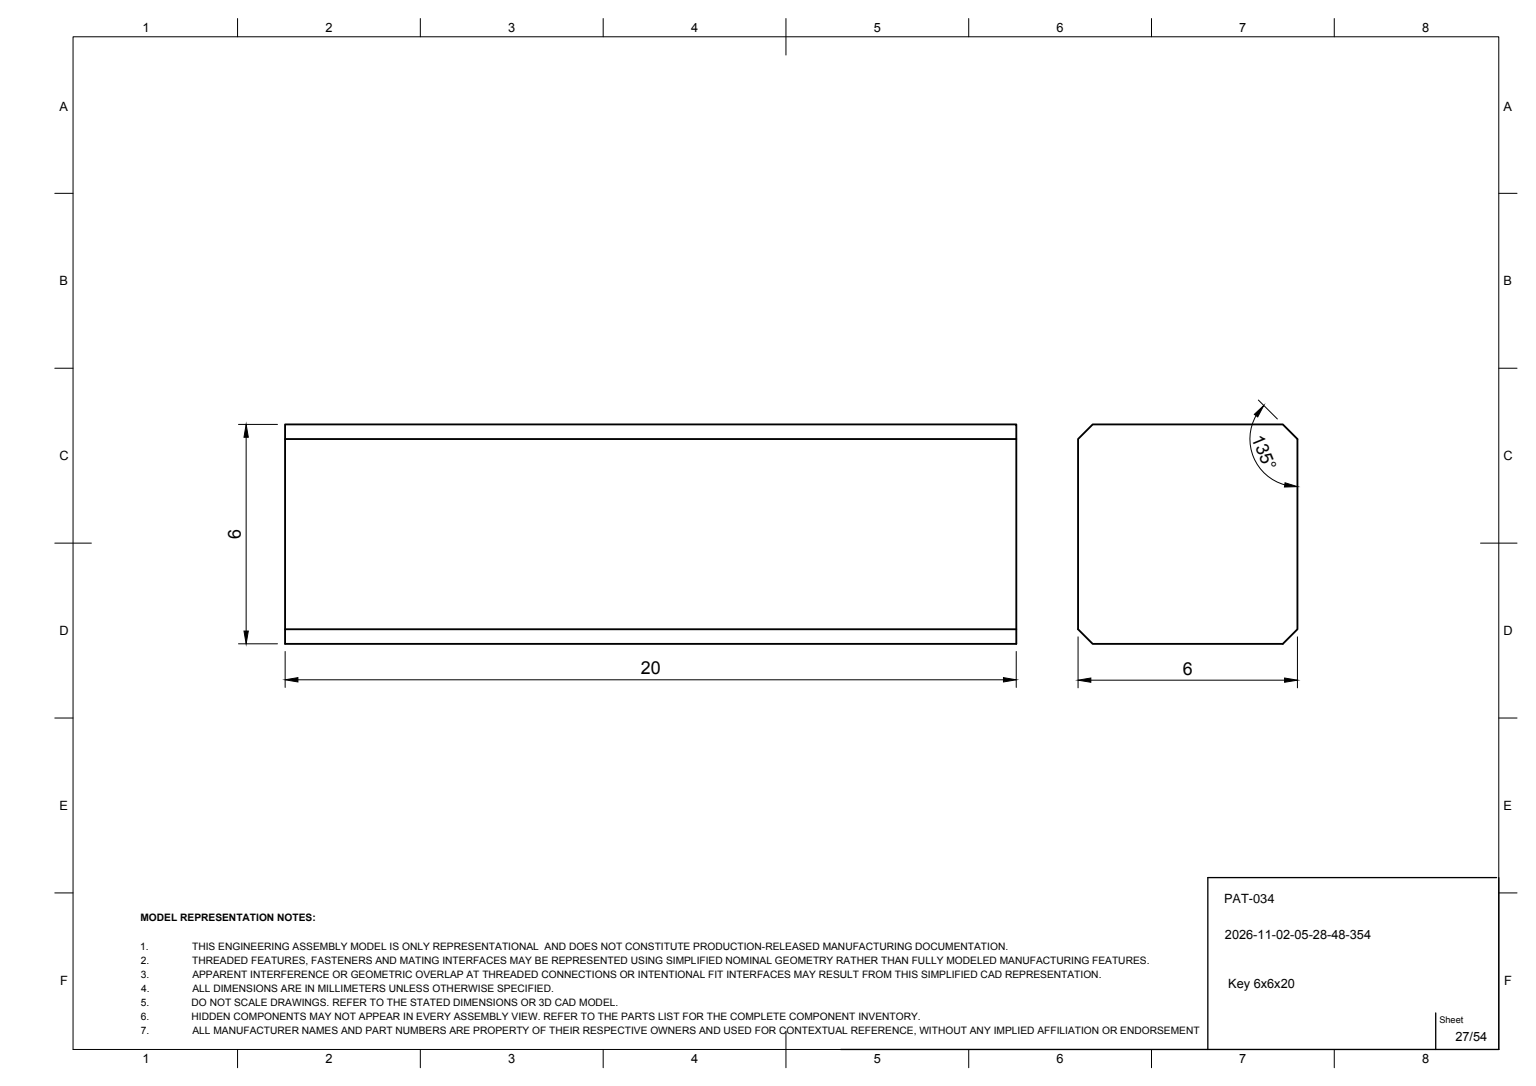
ISO-10303-21;
HEADER;
/* Generated by software containing ST-Developer
 * from STEP Tools, Inc. (www.steptools.com) 
 */

FILE_DESCRIPTION(
/* description */ ('Fatigue rig crank-slider'),
/* implementation_level */ '2;1');

FILE_NAME(
/* name */ 'Key 6x6x20.step',
/* time_stamp */ '2026-10-28T03:24:50-07:00',
/* author */ (''),
/* organization */ (''),
/* preprocessor_version */ 'ST-DEVELOPER v20.2',
/* originating_system */ 'Autodesk Translation Framework v15.17.0.0',
/* authorisation */ '');

FILE_SCHEMA (('AUTOMOTIVE_DESIGN { 1 0 10303 214 3 1 1 }'));
ENDSEC;

DATA;
#10=MECHANICAL_DESIGN_GEOMETRIC_PRESENTATION_REPRESENTATION('',(#613),#16911);
#512=SHAPE_REPRESENTATION_RELATIONSHIP('SRR','None',#17153,#562);
#562=ADVANCED_BREP_SHAPE_REPRESENTATION('',(#670),#16882);
#613=STYLED_ITEM('',(#17487),#670);
#670=MANIFOLD_SOLID_BREP('Body1',#8906);
#1063=PLANE('',#10025);
#1064=PLANE('',#10026);
#1065=PLANE('',#10027);
#1066=PLANE('',#10028);
#1067=PLANE('',#10029);
#1068=PLANE('',#10030);
#1069=PLANE('',#10031);
#1070=PLANE('',#10032);
#1071=PLANE('',#10033);
#1072=PLANE('',#10034);
#1496=FACE_OUTER_BOUND('',#2160,.T.);
#1497=FACE_OUTER_BOUND('',#2161,.T.);
#1498=FACE_OUTER_BOUND('',#2162,.T.);
#1499=FACE_OUTER_BOUND('',#2163,.T.);
#1500=FACE_OUTER_BOUND('',#2164,.T.);
#1501=FACE_OUTER_BOUND('',#2165,.T.);
#1502=FACE_OUTER_BOUND('',#2166,.T.);
#1503=FACE_OUTER_BOUND('',#2167,.T.);
#1504=FACE_OUTER_BOUND('',#2168,.T.);
#1505=FACE_OUTER_BOUND('',#2169,.T.);
#2160=EDGE_LOOP('',(#7158,#7159,#7160,#7161,#7162,#7163,#7164,#7165));
#2161=EDGE_LOOP('',(#7166,#7167,#7168,#7169));
#2162=EDGE_LOOP('',(#7170,#7171,#7172,#7173));
#2163=EDGE_LOOP('',(#7174,#7175,#7176,#7177));
#2164=EDGE_LOOP('',(#7178,#7179,#7180,#7181));
#2165=EDGE_LOOP('',(#7182,#7183,#7184,#7185,#7186,#7187,#7188,#7189));
#2166=EDGE_LOOP('',(#7190,#7191,#7192,#7193));
#2167=EDGE_LOOP('',(#7194,#7195,#7196,#7197));
#2168=EDGE_LOOP('',(#7198,#7199,#7200,#7201));
#2169=EDGE_LOOP('',(#7202,#7203,#7204,#7205));
#2784=LINE('',#15227,#3430);
#2785=LINE('',#15229,#3431);
#2786=LINE('',#15231,#3432);
#2787=LINE('',#15233,#3433);
#2788=LINE('',#15235,#3434);
#2789=LINE('',#15237,#3435);
#2790=LINE('',#15239,#3436);
#2791=LINE('',#15240,#3437);
#2792=LINE('',#15243,#3438);
#2793=LINE('',#15245,#3439);
#2794=LINE('',#15246,#3440);
#2795=LINE('',#15249,#3441);
#2796=LINE('',#15250,#3442);
#2797=LINE('',#15253,#3443);
#2798=LINE('',#15254,#3444);
#2799=LINE('',#15257,#3445);
#2800=LINE('',#15258,#3446);
#2801=LINE('',#15262,#3447);
#2802=LINE('',#15263,#3448);
#2803=LINE('',#15265,#3449);
#2804=LINE('',#15266,#3450);
#2805=LINE('',#15268,#3451);
#2806=LINE('',#15270,#3452);
#2807=LINE('',#15272,#3453);
#3430=VECTOR('',#11956,1.);
#3431=VECTOR('',#11957,1.);
#3432=VECTOR('',#11958,1.);
#3433=VECTOR('',#11959,1.);
#3434=VECTOR('',#11960,1.);
#3435=VECTOR('',#11961,1.);
#3436=VECTOR('',#11962,1.);
#3437=VECTOR('',#11963,1.);
#3438=VECTOR('',#11966,1.);
#3439=VECTOR('',#11967,1.);
#3440=VECTOR('',#11968,1.);
#3441=VECTOR('',#11971,1.);
#3442=VECTOR('',#11972,1.);
#3443=VECTOR('',#11975,1.);
#3444=VECTOR('',#11976,1.);
#3445=VECTOR('',#11979,1.);
#3446=VECTOR('',#11980,1.);
#3447=VECTOR('',#11983,1.);
#3448=VECTOR('',#11984,1.);
#3449=VECTOR('',#11985,1.);
#3450=VECTOR('',#11986,1.);
#3451=VECTOR('',#11989,1.);
#3452=VECTOR('',#11992,1.);
#3453=VECTOR('',#11995,1.);
#4545=VERTEX_POINT('',#15225);
#4546=VERTEX_POINT('',#15226);
#4547=VERTEX_POINT('',#15228);
#4548=VERTEX_POINT('',#15230);
#4549=VERTEX_POINT('',#15232);
#4550=VERTEX_POINT('',#15234);
#4551=VERTEX_POINT('',#15236);
#4552=VERTEX_POINT('',#15238);
#4553=VERTEX_POINT('',#15242);
#4554=VERTEX_POINT('',#15244);
#4555=VERTEX_POINT('',#15248);
#4556=VERTEX_POINT('',#15252);
#4557=VERTEX_POINT('',#15256);
#4558=VERTEX_POINT('',#15260);
#4559=VERTEX_POINT('',#15261);
#4560=VERTEX_POINT('',#15264);
#5477=EDGE_CURVE('',#4545,#4546,#2784,.T.);
#5478=EDGE_CURVE('',#4547,#4545,#2785,.T.);
#5479=EDGE_CURVE('',#4548,#4547,#2786,.T.);
#5480=EDGE_CURVE('',#4549,#4548,#2787,.T.);
#5481=EDGE_CURVE('',#4550,#4549,#2788,.T.);
#5482=EDGE_CURVE('',#4551,#4550,#2789,.T.);
#5483=EDGE_CURVE('',#4552,#4551,#2790,.T.);
#5484=EDGE_CURVE('',#4546,#4552,#2791,.T.);
#5485=EDGE_CURVE('',#4549,#4553,#2792,.T.);
#5486=EDGE_CURVE('',#4553,#4554,#2793,.T.);
#5487=EDGE_CURVE('',#4554,#4550,#2794,.T.);
#5488=EDGE_CURVE('',#4555,#4548,#2795,.T.);
#5489=EDGE_CURVE('',#4555,#4553,#2796,.T.);
#5490=EDGE_CURVE('',#4547,#4556,#2797,.T.);
#5491=EDGE_CURVE('',#4556,#4555,#2798,.T.);
#5492=EDGE_CURVE('',#4557,#4545,#2799,.T.);
#5493=EDGE_CURVE('',#4557,#4556,#2800,.T.);
#5494=EDGE_CURVE('',#4558,#4559,#2801,.T.);
#5495=EDGE_CURVE('',#4554,#4558,#2802,.T.);
#5496=EDGE_CURVE('',#4560,#4557,#2803,.T.);
#5497=EDGE_CURVE('',#4559,#4560,#2804,.T.);
#5498=EDGE_CURVE('',#4551,#4558,#2805,.T.);
#5499=EDGE_CURVE('',#4546,#4560,#2806,.T.);
#5500=EDGE_CURVE('',#4559,#4552,#2807,.T.);
#7158=ORIENTED_EDGE('',*,*,#5477,.F.);
#7159=ORIENTED_EDGE('',*,*,#5478,.F.);
#7160=ORIENTED_EDGE('',*,*,#5479,.F.);
#7161=ORIENTED_EDGE('',*,*,#5480,.F.);
#7162=ORIENTED_EDGE('',*,*,#5481,.F.);
#7163=ORIENTED_EDGE('',*,*,#5482,.F.);
#7164=ORIENTED_EDGE('',*,*,#5483,.F.);
#7165=ORIENTED_EDGE('',*,*,#5484,.F.);
#7166=ORIENTED_EDGE('',*,*,#5481,.T.);
#7167=ORIENTED_EDGE('',*,*,#5485,.T.);
#7168=ORIENTED_EDGE('',*,*,#5486,.T.);
#7169=ORIENTED_EDGE('',*,*,#5487,.T.);
#7170=ORIENTED_EDGE('',*,*,#5480,.T.);
#7171=ORIENTED_EDGE('',*,*,#5488,.F.);
#7172=ORIENTED_EDGE('',*,*,#5489,.T.);
#7173=ORIENTED_EDGE('',*,*,#5485,.F.);
#7174=ORIENTED_EDGE('',*,*,#5479,.T.);
#7175=ORIENTED_EDGE('',*,*,#5490,.T.);
#7176=ORIENTED_EDGE('',*,*,#5491,.T.);
#7177=ORIENTED_EDGE('',*,*,#5488,.T.);
#7178=ORIENTED_EDGE('',*,*,#5478,.T.);
#7179=ORIENTED_EDGE('',*,*,#5492,.F.);
#7180=ORIENTED_EDGE('',*,*,#5493,.T.);
#7181=ORIENTED_EDGE('',*,*,#5490,.F.);
#7182=ORIENTED_EDGE('',*,*,#5494,.F.);
#7183=ORIENTED_EDGE('',*,*,#5495,.F.);
#7184=ORIENTED_EDGE('',*,*,#5486,.F.);
#7185=ORIENTED_EDGE('',*,*,#5489,.F.);
#7186=ORIENTED_EDGE('',*,*,#5491,.F.);
#7187=ORIENTED_EDGE('',*,*,#5493,.F.);
#7188=ORIENTED_EDGE('',*,*,#5496,.F.);
#7189=ORIENTED_EDGE('',*,*,#5497,.F.);
#7190=ORIENTED_EDGE('',*,*,#5482,.T.);
#7191=ORIENTED_EDGE('',*,*,#5487,.F.);
#7192=ORIENTED_EDGE('',*,*,#5495,.T.);
#7193=ORIENTED_EDGE('',*,*,#5498,.F.);
#7194=ORIENTED_EDGE('',*,*,#5477,.T.);
#7195=ORIENTED_EDGE('',*,*,#5499,.T.);
#7196=ORIENTED_EDGE('',*,*,#5496,.T.);
#7197=ORIENTED_EDGE('',*,*,#5492,.T.);
#7198=ORIENTED_EDGE('',*,*,#5483,.T.);
#7199=ORIENTED_EDGE('',*,*,#5498,.T.);
#7200=ORIENTED_EDGE('',*,*,#5494,.T.);
#7201=ORIENTED_EDGE('',*,*,#5500,.T.);
#7202=ORIENTED_EDGE('',*,*,#5484,.T.);
#7203=ORIENTED_EDGE('',*,*,#5500,.F.);
#7204=ORIENTED_EDGE('',*,*,#5497,.T.);
#7205=ORIENTED_EDGE('',*,*,#5499,.F.);
#8634=ADVANCED_FACE('',(#1496),#1063,.F.);
#8635=ADVANCED_FACE('',(#1497),#1064,.T.);
#8636=ADVANCED_FACE('',(#1498),#1065,.T.);
#8637=ADVANCED_FACE('',(#1499),#1066,.T.);
#8638=ADVANCED_FACE('',(#1500),#1067,.T.);
#8639=ADVANCED_FACE('',(#1501),#1068,.T.);
#8640=ADVANCED_FACE('',(#1502),#1069,.F.);
#8641=ADVANCED_FACE('',(#1503),#1070,.T.);
#8642=ADVANCED_FACE('',(#1504),#1071,.T.);
#8643=ADVANCED_FACE('',(#1505),#1072,.T.);
#8906=CLOSED_SHELL('',(#8634,#8635,#8636,#8637,#8638,#8639,#8640,#8641,
#8642,#8643));
#10024=AXIS2_PLACEMENT_3D('',#15223,#11952,#11953);
#10025=AXIS2_PLACEMENT_3D('',#15224,#11954,#11955);
#10026=AXIS2_PLACEMENT_3D('',#15241,#11964,#11965);
#10027=AXIS2_PLACEMENT_3D('',#15247,#11969,#11970);
#10028=AXIS2_PLACEMENT_3D('',#15251,#11973,#11974);
#10029=AXIS2_PLACEMENT_3D('',#15255,#11977,#11978);
#10030=AXIS2_PLACEMENT_3D('',#15259,#11981,#11982);
#10031=AXIS2_PLACEMENT_3D('',#15267,#11987,#11988);
#10032=AXIS2_PLACEMENT_3D('',#15269,#11990,#11991);
#10033=AXIS2_PLACEMENT_3D('',#15271,#11993,#11994);
#10034=AXIS2_PLACEMENT_3D('',#15273,#11996,#11997);
#11952=DIRECTION('axis',(0.,0.,1.));
#11953=DIRECTION('refdir',(1.,0.,0.));
#11954=DIRECTION('center_axis',(1.,0.,0.));
#11955=DIRECTION('ref_axis',(0.,0.,-1.));
#11956=DIRECTION('',(0.,-0.707106781186547,-0.707106781186548));
#11957=DIRECTION('',(0.,-1.,0.));
#11958=DIRECTION('',(0.,-0.707106781186547,0.707106781186548));
#11959=DIRECTION('',(0.,0.,1.));
#11960=DIRECTION('',(0.,0.707106781186547,0.707106781186548));
#11961=DIRECTION('',(0.,1.,0.));
#11962=DIRECTION('',(0.,0.707106781186547,-0.707106781186548));
#11963=DIRECTION('',(0.,0.,-1.));
#11964=DIRECTION('center_axis',(0.,0.707106781186548,-0.707106781186547));
#11965=DIRECTION('ref_axis',(-1.,0.,0.));
#11966=DIRECTION('',(1.,0.,0.));
#11967=DIRECTION('',(0.,-0.707106781186547,-0.707106781186548));
#11968=DIRECTION('',(-1.,0.,0.));
#11969=DIRECTION('center_axis',(0.,1.,0.));
#11970=DIRECTION('ref_axis',(-1.,0.,0.));
#11971=DIRECTION('',(-1.,0.,0.));
#11972=DIRECTION('',(0.,0.,-1.));
#11973=DIRECTION('center_axis',(0.,0.707106781186548,0.707106781186547));
#11974=DIRECTION('ref_axis',(1.,0.,0.));
#11975=DIRECTION('',(1.,0.,0.));
#11976=DIRECTION('',(0.,0.707106781186547,-0.707106781186548));
#11977=DIRECTION('center_axis',(0.,0.,1.));
#11978=DIRECTION('ref_axis',(1.,0.,0.));
#11979=DIRECTION('',(-1.,0.,0.));
#11980=DIRECTION('',(0.,1.,0.));
#11981=DIRECTION('center_axis',(1.,0.,0.));
#11982=DIRECTION('ref_axis',(0.,0.,-1.));
#11983=DIRECTION('',(0.,-0.707106781186547,0.707106781186548));
#11984=DIRECTION('',(0.,-1.,0.));
#11985=DIRECTION('',(0.,0.707106781186547,0.707106781186548));
#11986=DIRECTION('',(0.,0.,1.));
#11987=DIRECTION('center_axis',(0.,0.,1.));
#11988=DIRECTION('ref_axis',(1.,0.,0.));
#11989=DIRECTION('',(1.,0.,0.));
#11990=DIRECTION('center_axis',(0.,-0.707106781186548,0.707106781186547));
#11991=DIRECTION('ref_axis',(1.,0.,0.));
#11992=DIRECTION('',(1.,0.,0.));
#11993=DIRECTION('center_axis',(0.,-0.707106781186548,-0.707106781186547));
#11994=DIRECTION('ref_axis',(-1.,0.,0.));
#11995=DIRECTION('',(-1.,0.,0.));
#11996=DIRECTION('center_axis',(0.,-1.,0.));
#11997=DIRECTION('ref_axis',(1.,0.,0.));
#15223=CARTESIAN_POINT('',(0.,0.,0.));
#15224=CARTESIAN_POINT('Origin',(-1.,0.,0.35));
#15225=CARTESIAN_POINT('',(-1.,-0.26,0.6));
#15226=CARTESIAN_POINT('',(-1.,-0.3,0.56));
#15227=CARTESIAN_POINT('',(-1.,-0.2675,0.5925));
#15228=CARTESIAN_POINT('',(-1.,0.26,0.6));
#15229=CARTESIAN_POINT('',(-1.,0.,0.6));
#15230=CARTESIAN_POINT('',(-1.,0.3,0.56));
#15231=CARTESIAN_POINT('',(-1.,0.2675,0.5925));
#15232=CARTESIAN_POINT('',(-1.,0.3,0.04));
#15233=CARTESIAN_POINT('',(-1.,0.3,0.175));
#15234=CARTESIAN_POINT('',(-1.,0.26,0.));
#15235=CARTESIAN_POINT('',(-1.,0.2925,0.0325));
#15236=CARTESIAN_POINT('',(-1.,-0.26,0.));
#15237=CARTESIAN_POINT('',(-1.,0.,0.));
#15238=CARTESIAN_POINT('',(-1.,-0.3,0.04));
#15239=CARTESIAN_POINT('',(-1.,-0.2925,0.0325));
#15240=CARTESIAN_POINT('',(-1.,-0.3,0.175));
#15241=CARTESIAN_POINT('Origin',(0.75,0.28,0.02));
#15242=CARTESIAN_POINT('',(1.,0.3,0.04));
#15243=CARTESIAN_POINT('',(0.75,0.3,0.04));
#15244=CARTESIAN_POINT('',(1.,0.26,0.));
#15245=CARTESIAN_POINT('',(1.,0.2925,0.0325));
#15246=CARTESIAN_POINT('',(0.75,0.26,0.));
#15247=CARTESIAN_POINT('Origin',(1.5,0.3,0.));
#15248=CARTESIAN_POINT('',(1.,0.3,0.56));
#15249=CARTESIAN_POINT('',(0.75,0.3,0.56));
#15250=CARTESIAN_POINT('',(1.,0.3,0.175));
#15251=CARTESIAN_POINT('Origin',(0.75,0.28,0.58));
#15252=CARTESIAN_POINT('',(1.,0.26,0.6));
#15253=CARTESIAN_POINT('',(0.75,0.26,0.6));
#15254=CARTESIAN_POINT('',(1.,0.2675,0.5925));
#15255=CARTESIAN_POINT('Origin',(0.,0.,0.6));
#15256=CARTESIAN_POINT('',(1.,-0.26,0.6));
#15257=CARTESIAN_POINT('',(-0.75,-0.26,0.6));
#15258=CARTESIAN_POINT('',(1.,0.,0.6));
#15259=CARTESIAN_POINT('Origin',(1.,0.,0.35));
#15260=CARTESIAN_POINT('',(1.,-0.26,0.));
#15261=CARTESIAN_POINT('',(1.,-0.3,0.04));
#15262=CARTESIAN_POINT('',(1.,-0.2925,0.0325));
#15263=CARTESIAN_POINT('',(1.,0.,0.));
#15264=CARTESIAN_POINT('',(1.,-0.3,0.56));
#15265=CARTESIAN_POINT('',(1.,-0.2675,0.5925));
#15266=CARTESIAN_POINT('',(1.,-0.3,0.175));
#15267=CARTESIAN_POINT('Origin',(0.,0.,0.));
#15268=CARTESIAN_POINT('',(-0.75,-0.26,0.));
#15269=CARTESIAN_POINT('Origin',(-0.75,-0.28,0.58));
#15270=CARTESIAN_POINT('',(-0.75,-0.3,0.56));
#15271=CARTESIAN_POINT('Origin',(-0.75,-0.28,0.02));
#15272=CARTESIAN_POINT('',(-0.75,-0.3,0.04));
#15273=CARTESIAN_POINT('Origin',(-1.5,-0.3,0.));
#16823=UNCERTAINTY_MEASURE_WITH_UNIT(LENGTH_MEASURE(0.001),#16912,
'DISTANCE_ACCURACY_VALUE',
'Maximum model space distance between geometric entities at asserted c
onnectivities');
#16852=UNCERTAINTY_MEASURE_WITH_UNIT(LENGTH_MEASURE(0.001),#16912,
'DISTANCE_ACCURACY_VALUE',
'Maximum model space distance between geometric entities at asserted c
onnectivities');
#16882=(
GEOMETRIC_REPRESENTATION_CONTEXT(3)
GLOBAL_UNCERTAINTY_ASSIGNED_CONTEXT((#16823))
GLOBAL_UNIT_ASSIGNED_CONTEXT((#16912,#16914,#16915))
REPRESENTATION_CONTEXT('','3D')
);
#16911=(
GEOMETRIC_REPRESENTATION_CONTEXT(3)
GLOBAL_UNCERTAINTY_ASSIGNED_CONTEXT((#16852))
GLOBAL_UNIT_ASSIGNED_CONTEXT((#16912,#16914,#16915))
REPRESENTATION_CONTEXT('','3D')
);
#16912=(
LENGTH_UNIT()
NAMED_UNIT(*)
SI_UNIT(.CENTI.,.METRE.)
);
#16914=(
NAMED_UNIT(*)
PLANE_ANGLE_UNIT()
SI_UNIT($,.RADIAN.)
);
#16915=(
NAMED_UNIT(*)
SI_UNIT($,.STERADIAN.)
SOLID_ANGLE_UNIT()
);
#16945=SHAPE_DEFINITION_REPRESENTATION(#17005,#17153);
#17005=PRODUCT_DEFINITION_SHAPE('',$,#17212);
#17153=SHAPE_REPRESENTATION('',(#10024),#16882);
#17182=PRODUCT_DEFINITION_CONTEXT('part definition',#17358,'design');
#17212=PRODUCT_DEFINITION('Key 6x6x20','Key 6x6x20',#17270,#17182);
#17270=PRODUCT_DEFINITION_FORMATION('',$,#17389);
#17358=APPLICATION_CONTEXT(
'Core Data for Automotive Mechanical Design Process');
#17359=PRODUCT_CONTEXT('part definition',#17358,'mechanical');
#17389=PRODUCT('Key 6x6x20','Key 6x6x20','Key 6x6x20',(#17359));
#17481=COLOUR_RGB('Grey',0.48,0.52,0.57);
#17482=FILL_AREA_STYLE_COLOUR('',#17481);
#17483=FILL_AREA_STYLE('',(#17482));
#17484=SURFACE_STYLE_FILL_AREA(#17483);
#17485=SURFACE_SIDE_STYLE('',(#17484));
#17486=SURFACE_STYLE_USAGE(.BOTH.,#17485);
#17487=PRESENTATION_STYLE_ASSIGNMENT((#17486));
ENDSEC;
END-ISO-10303-21;
